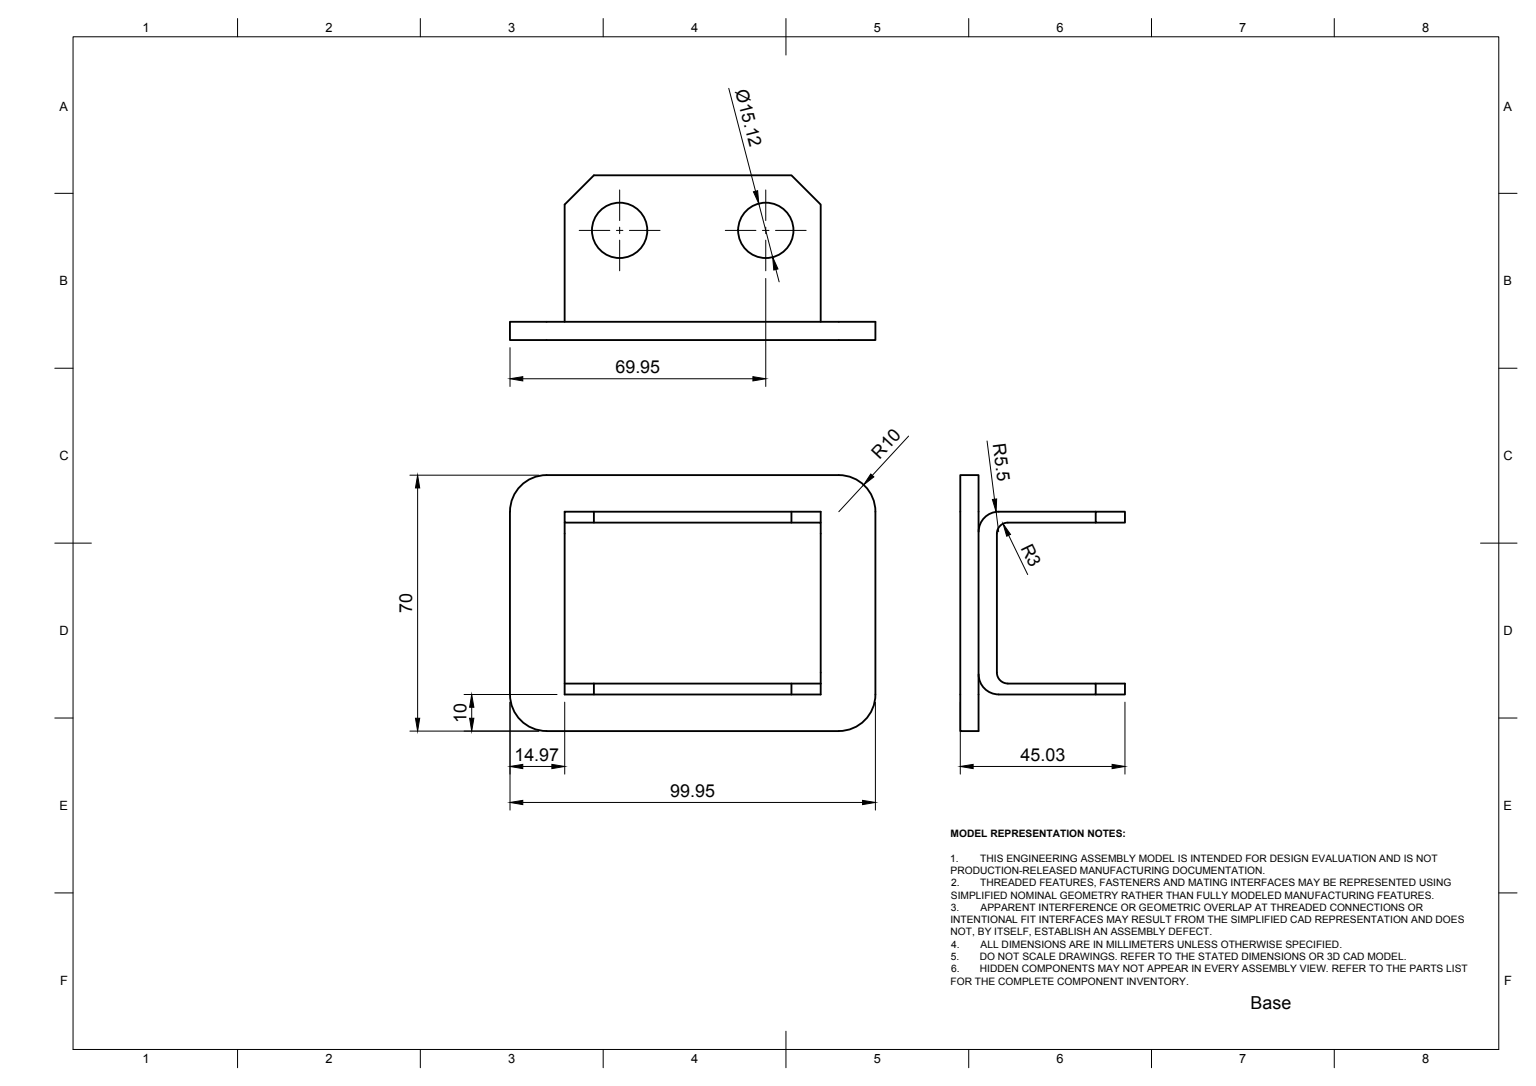
ISO-10303-21;
HEADER;
/* Generated by software containing ST-Developer
 * from STEP Tools, Inc. (www.steptools.com) 
 */

FILE_DESCRIPTION(
/* description */ (''),
/* implementation_level */ '2;1');

FILE_NAME(
/* name */ 'Base.step',
/* time_stamp */ '2026-10-06T13:41:14-07:00',
/* author */ (''),
/* organization */ (''),
/* preprocessor_version */ 'ST-DEVELOPER v20.2',
/* originating_system */ 'Autodesk Translation Framework v15.15.0.0',
/* authorisation */ '');

FILE_SCHEMA (('AUTOMOTIVE_DESIGN { 1 0 10303 214 3 1 1 }'));
ENDSEC;

DATA;
#10=MECHANICAL_DESIGN_GEOMETRIC_PRESENTATION_REPRESENTATION('',(#1960),#279266);
#1942=SHAPE_REPRESENTATION_RELATIONSHIP('SRR','None',#279301,#1951);
#1951=ADVANCED_BREP_SHAPE_REPRESENTATION('',(#1969),#279257);
#1960=STYLED_ITEM('',(#279355),#1969);
#1969=MANIFOLD_SOLID_BREP('Body1',#14938);
#1978=FACE_BOUND('',#2587,.T.);
#1979=FACE_BOUND('',#2588,.T.);
#1980=FACE_BOUND('',#2591,.T.);
#1981=FACE_BOUND('',#2592,.T.);
#1982=FACE_BOUND('',#2604,.T.);
#1983=FACE_BOUND('',#2609,.T.);
#1984=FACE_BOUND('',#2610,.T.);
#1985=FACE_BOUND('',#2613,.T.);
#1986=FACE_BOUND('',#2614,.T.);
#2024=PLANE('',#15055);
#2025=PLANE('',#15059);
#2026=PLANE('',#15063);
#2027=PLANE('',#15068);
#2028=PLANE('',#15071);
#2029=PLANE('',#15072);
#2030=PLANE('',#15076);
#2031=PLANE('',#15077);
#2032=PLANE('',#15083);
#2033=PLANE('',#15087);
#2034=PLANE('',#15088);
#2035=PLANE('',#15089);
#2036=PLANE('',#15090);
#2037=PLANE('',#15093);
#2038=PLANE('',#15097);
#2039=PLANE('',#15099);
#2040=PLANE('',#15101);
#2041=PLANE('',#15102);
#2042=PLANE('',#15103);
#2110=FACE_OUTER_BOUND('',#2580,.T.);
#2111=FACE_OUTER_BOUND('',#2581,.T.);
#2112=FACE_OUTER_BOUND('',#2582,.T.);
#2113=FACE_OUTER_BOUND('',#2583,.T.);
#2114=FACE_OUTER_BOUND('',#2584,.T.);
#2115=FACE_OUTER_BOUND('',#2585,.T.);
#2116=FACE_OUTER_BOUND('',#2586,.T.);
#2117=FACE_OUTER_BOUND('',#2589,.T.);
#2118=FACE_OUTER_BOUND('',#2590,.T.);
#2119=FACE_OUTER_BOUND('',#2593,.T.);
#2120=FACE_OUTER_BOUND('',#2594,.T.);
#2121=FACE_OUTER_BOUND('',#2595,.T.);
#2122=FACE_OUTER_BOUND('',#2596,.T.);
#2123=FACE_OUTER_BOUND('',#2597,.T.);
#2124=FACE_OUTER_BOUND('',#2598,.T.);
#2125=FACE_OUTER_BOUND('',#2599,.T.);
#2126=FACE_OUTER_BOUND('',#2600,.T.);
#2127=FACE_OUTER_BOUND('',#2601,.T.);
#2128=FACE_OUTER_BOUND('',#2602,.T.);
#2129=FACE_OUTER_BOUND('',#2603,.T.);
#2130=FACE_OUTER_BOUND('',#2605,.T.);
#2131=FACE_OUTER_BOUND('',#2606,.T.);
#2132=FACE_OUTER_BOUND('',#2607,.T.);
#2133=FACE_OUTER_BOUND('',#2608,.T.);
#2134=FACE_OUTER_BOUND('',#2611,.T.);
#2135=FACE_OUTER_BOUND('',#2612,.T.);
#2136=FACE_OUTER_BOUND('',#2615,.T.);
#2137=FACE_OUTER_BOUND('',#2616,.T.);
#2138=FACE_OUTER_BOUND('',#2617,.T.);
#2139=FACE_OUTER_BOUND('',#2618,.T.);
#2140=FACE_OUTER_BOUND('',#2619,.T.);
#2580=EDGE_LOOP('',(#8972,#8973,#8974,#8975));
#2581=EDGE_LOOP('',(#8976,#8977,#8978,#8979));
#2582=EDGE_LOOP('',(#8980,#8981,#8982,#8983));
#2583=EDGE_LOOP('',(#8984,#8985,#8986,#8987));
#2584=EDGE_LOOP('',(#8988,#8989,#8990,#8991));
#2585=EDGE_LOOP('',(#8992,#8993,#8994,#8995));
#2586=EDGE_LOOP('',(#8996,#8997,#8998,#8999,#9000,#9001));
#2587=EDGE_LOOP('',(#9002));
#2588=EDGE_LOOP('',(#9003));
#2589=EDGE_LOOP('',(#9004,#9005,#9006,#9007));
#2590=EDGE_LOOP('',(#9008,#9009,#9010,#9011,#9012,#9013));
#2591=EDGE_LOOP('',(#9014));
#2592=EDGE_LOOP('',(#9015));
#2593=EDGE_LOOP('',(#9016,#9017,#9018,#9019));
#2594=EDGE_LOOP('',(#9020,#9021,#9022,#9023));
#2595=EDGE_LOOP('',(#9024,#9025,#9026,#9027));
#2596=EDGE_LOOP('',(#9028,#9029,#9030,#9031));
#2597=EDGE_LOOP('',(#9032,#9033,#9034,#9035));
#2598=EDGE_LOOP('',(#9036,#9037,#9038,#9039,#9040,#9041,#9042,#9043,#9044,
#9045,#9046,#9047));
#2599=EDGE_LOOP('',(#9048,#9049,#9050,#9051));
#2600=EDGE_LOOP('',(#9052,#9053,#9054,#9055));
#2601=EDGE_LOOP('',(#9056,#9057,#9058,#9059));
#2602=EDGE_LOOP('',(#9060,#9061,#9062,#9063));
#2603=EDGE_LOOP('',(#9064,#9065,#9066,#9067,#9068,#9069,#9070,#9071));
#2604=EDGE_LOOP('',(#9072,#9073,#9074,#9075));
#2605=EDGE_LOOP('',(#9076,#9077,#9078,#9079));
#2606=EDGE_LOOP('',(#9080,#9081,#9082,#9083,#9084,#9085,#9086,#9087));
#2607=EDGE_LOOP('',(#9088,#9089,#9090,#9091));
#2608=EDGE_LOOP('',(#9092,#9093,#9094,#9095,#9096,#9097));
#2609=EDGE_LOOP('',(#9098));
#2610=EDGE_LOOP('',(#9099));
#2611=EDGE_LOOP('',(#9100,#9101,#9102,#9103));
#2612=EDGE_LOOP('',(#9104,#9105,#9106,#9107,#9108,#9109));
#2613=EDGE_LOOP('',(#9110));
#2614=EDGE_LOOP('',(#9111));
#2615=EDGE_LOOP('',(#9112,#9113,#9114,#9115,#9116,#9117,#9118,#9119,#9120,
#9121,#9122,#9123));
#2616=EDGE_LOOP('',(#9124,#9125,#9126,#9127));
#2617=EDGE_LOOP('',(#9128,#9129,#9130,#9131));
#2618=EDGE_LOOP('',(#9132,#9133,#9134,#9135));
#2619=EDGE_LOOP('',(#9136,#9137,#9138,#9139));
#3096=LINE('',#17463,#3624);
#3097=LINE('',#17466,#3625);
#3098=LINE('',#17471,#3626);
#3099=LINE('',#17476,#3627);
#3100=LINE('',#17478,#3628);
#3101=LINE('',#17480,#3629);
#3102=LINE('',#17481,#3630);
#3103=LINE('',#17487,#3631);
#3104=LINE('',#17490,#3632);
#3105=LINE('',#17492,#3633);
#3106=LINE('',#17493,#3634);
#3107=LINE('',#17497,#3635);
#3108=LINE('',#17501,#3636);
#3109=LINE('',#17505,#3637);
#3110=LINE('',#17507,#3638);
#3111=LINE('',#17508,#3639);
#3112=LINE('',#17509,#3640);
#3113=LINE('',#17517,#3641);
#3114=LINE('',#17520,#3642);
#3115=LINE('',#17522,#3643);
#3116=LINE('',#17524,#3644);
#3117=LINE('',#17526,#3645);
#3118=LINE('',#17527,#3646);
#3119=LINE('',#17531,#3647);
#3120=LINE('',#17533,#3648);
#3121=LINE('',#17535,#3649);
#3122=LINE('',#17541,#3650);
#3123=LINE('',#17544,#3651);
#3124=LINE('',#17546,#3652);
#3125=LINE('',#17547,#3653);
#3126=LINE('',#17553,#3654);
#3127=LINE('',#17555,#3655);
#3128=LINE('',#17557,#3656);
#3129=LINE('',#17560,#3657);
#3130=LINE('',#17561,#3658);
#3131=LINE('',#17566,#3659);
#3132=LINE('',#17570,#3660);
#3133=LINE('',#17572,#3661);
#3134=LINE('',#17573,#3662);
#3135=LINE('',#17579,#3663);
#3136=LINE('',#17582,#3664);
#3137=LINE('',#17584,#3665);
#3138=LINE('',#17585,#3666);
#3139=LINE('',#17587,#3667);
#3140=LINE('',#17589,#3668);
#3141=LINE('',#17590,#3669);
#3142=LINE('',#17592,#3670);
#3143=LINE('',#17596,#3671);
#3144=LINE('',#17599,#3672);
#3145=LINE('',#17602,#3673);
#3146=LINE('',#17604,#3674);
#3147=LINE('',#17605,#3675);
#3148=LINE('',#17611,#3676);
#3149=LINE('',#17614,#3677);
#3150=LINE('',#17616,#3678);
#3151=LINE('',#17617,#3679);
#3152=LINE('',#17621,#3680);
#3153=LINE('',#17622,#3681);
#3154=LINE('',#17624,#3682);
#3155=LINE('',#17626,#3683);
#3624=VECTOR('',#15682,10.);
#3625=VECTOR('',#15685,10.);
#3626=VECTOR('',#15690,7.55784864301595);
#3627=VECTOR('',#15695,10.);
#3628=VECTOR('',#15696,10.);
#3629=VECTOR('',#15697,9.99999999999999);
#3630=VECTOR('',#15698,10.);
#3631=VECTOR('',#15703,10.);
#3632=VECTOR('',#15706,10.);
#3633=VECTOR('',#15709,10.);
#3634=VECTOR('',#15710,10.);
#3635=VECTOR('',#15713,10.);
#3636=VECTOR('',#15716,10.);
#3637=VECTOR('',#15721,10.);
#3638=VECTOR('',#15722,10.);
#3639=VECTOR('',#15723,10.);
#3640=VECTOR('',#15724,10.);
#3641=VECTOR('',#15731,10.);
#3642=VECTOR('',#15734,10.);
#3643=VECTOR('',#15737,10.);
#3644=VECTOR('',#15738,10.);
#3645=VECTOR('',#15739,9.99999999999999);
#3646=VECTOR('',#15740,10.);
#3647=VECTOR('',#15745,7.55784864301595);
#3648=VECTOR('',#15748,10.);
#3649=VECTOR('',#15751,10.);
#3650=VECTOR('',#15756,10.);
#3651=VECTOR('',#15759,10.);
#3652=VECTOR('',#15762,10.);
#3653=VECTOR('',#15763,10.);
#3654=VECTOR('',#15768,10.);
#3655=VECTOR('',#15769,10.);
#3656=VECTOR('',#15770,10.);
#3657=VECTOR('',#15773,10.);
#3658=VECTOR('',#15774,10.);
#3659=VECTOR('',#15779,7.55784864301595);
#3660=VECTOR('',#15784,10.);
#3661=VECTOR('',#15785,9.99999999999999);
#3662=VECTOR('',#15786,10.);
#3663=VECTOR('',#15791,10.);
#3664=VECTOR('',#15794,10.);
#3665=VECTOR('',#15797,10.);
#3666=VECTOR('',#15798,10.);
#3667=VECTOR('',#15801,10.);
#3668=VECTOR('',#15802,10.);
#3669=VECTOR('',#15803,10.);
#3670=VECTOR('',#15806,10.);
#3671=VECTOR('',#15811,10.);
#3672=VECTOR('',#15814,10.);
#3673=VECTOR('',#15817,10.);
#3674=VECTOR('',#15818,10.);
#3675=VECTOR('',#15819,10.);
#3676=VECTOR('',#15826,10.);
#3677=VECTOR('',#15829,10.);
#3678=VECTOR('',#15830,9.99999999999999);
#3679=VECTOR('',#15831,10.);
#3680=VECTOR('',#15836,10.);
#3681=VECTOR('',#15837,10.);
#3682=VECTOR('',#15840,7.55784864301595);
#3683=VECTOR('',#15843,10.);
#4152=CIRCLE('',#15050,10.);
#4153=CIRCLE('',#15051,10.);
#4154=CIRCLE('',#15053,7.55784864301595);
#4155=CIRCLE('',#15054,7.55784864301595);
#4156=CIRCLE('',#15057,10.);
#4157=CIRCLE('',#15058,10.);
#4158=CIRCLE('',#15061,3.);
#4159=CIRCLE('',#15062,3.);
#4160=CIRCLE('',#15064,7.55784864301595);
#4161=CIRCLE('',#15066,5.5);
#4162=CIRCLE('',#15067,5.5);
#4163=CIRCLE('',#15069,7.55784864301595);
#4164=CIRCLE('',#15074,10.);
#4165=CIRCLE('',#15075,10.);
#4166=CIRCLE('',#15078,5.5);
#4167=CIRCLE('',#15079,3.);
#4168=CIRCLE('',#15081,7.55784864301595);
#4169=CIRCLE('',#15082,7.55784864301595);
#4170=CIRCLE('',#15085,10.);
#4171=CIRCLE('',#15086,10.);
#4172=CIRCLE('',#15092,3.);
#4173=CIRCLE('',#15094,7.55784864301595);
#4174=CIRCLE('',#15096,5.5);
#4175=CIRCLE('',#15098,7.55784864301595);
#4300=VERTEX_POINT('',#17459);
#4301=VERTEX_POINT('',#17460);
#4302=VERTEX_POINT('',#17462);
#4303=VERTEX_POINT('',#17464);
#4304=VERTEX_POINT('',#17468);
#4305=VERTEX_POINT('',#17470);
#4306=VERTEX_POINT('',#17474);
#4307=VERTEX_POINT('',#17475);
#4308=VERTEX_POINT('',#17477);
#4309=VERTEX_POINT('',#17479);
#4310=VERTEX_POINT('',#17483);
#4311=VERTEX_POINT('',#17484);
#4312=VERTEX_POINT('',#17486);
#4313=VERTEX_POINT('',#17488);
#4314=VERTEX_POINT('',#17495);
#4315=VERTEX_POINT('',#17496);
#4316=VERTEX_POINT('',#17498);
#4317=VERTEX_POINT('',#17500);
#4318=VERTEX_POINT('',#17504);
#4319=VERTEX_POINT('',#17506);
#4320=VERTEX_POINT('',#17510);
#4321=VERTEX_POINT('',#17513);
#4322=VERTEX_POINT('',#17514);
#4323=VERTEX_POINT('',#17516);
#4324=VERTEX_POINT('',#17518);
#4325=VERTEX_POINT('',#17523);
#4326=VERTEX_POINT('',#17525);
#4327=VERTEX_POINT('',#17528);
#4328=VERTEX_POINT('',#17537);
#4329=VERTEX_POINT('',#17538);
#4330=VERTEX_POINT('',#17540);
#4331=VERTEX_POINT('',#17542);
#4332=VERTEX_POINT('',#17549);
#4333=VERTEX_POINT('',#17550);
#4334=VERTEX_POINT('',#17552);
#4335=VERTEX_POINT('',#17554);
#4336=VERTEX_POINT('',#17556);
#4337=VERTEX_POINT('',#17558);
#4338=VERTEX_POINT('',#17563);
#4339=VERTEX_POINT('',#17565);
#4340=VERTEX_POINT('',#17569);
#4341=VERTEX_POINT('',#17571);
#4342=VERTEX_POINT('',#17575);
#4343=VERTEX_POINT('',#17576);
#4344=VERTEX_POINT('',#17578);
#4345=VERTEX_POINT('',#17580);
#4346=VERTEX_POINT('',#17588);
#4347=VERTEX_POINT('',#17595);
#4348=VERTEX_POINT('',#17597);
#4349=VERTEX_POINT('',#17601);
#4350=VERTEX_POINT('',#17603);
#4351=VERTEX_POINT('',#17606);
#4352=VERTEX_POINT('',#17609);
#4353=VERTEX_POINT('',#17613);
#4354=VERTEX_POINT('',#17615);
#4355=VERTEX_POINT('',#17618);
#6411=EDGE_CURVE('',#4300,#4301,#4152,.T.);
#6412=EDGE_CURVE('',#4301,#4302,#3096,.T.);
#6413=EDGE_CURVE('',#4302,#4303,#4153,.T.);
#6414=EDGE_CURVE('',#4303,#4300,#3097,.T.);
#6415=EDGE_CURVE('',#4304,#4304,#4154,.T.);
#6416=EDGE_CURVE('',#4304,#4305,#3098,.T.);
#6417=EDGE_CURVE('',#4305,#4305,#4155,.T.);
#6418=EDGE_CURVE('',#4306,#4307,#3099,.T.);
#6419=EDGE_CURVE('',#4307,#4308,#3100,.T.);
#6420=EDGE_CURVE('',#4309,#4308,#3101,.T.);
#6421=EDGE_CURVE('',#4306,#4309,#3102,.T.);
#6422=EDGE_CURVE('',#4310,#4311,#4156,.T.);
#6423=EDGE_CURVE('',#4312,#4310,#3103,.T.);
#6424=EDGE_CURVE('',#4313,#4312,#4157,.T.);
#6425=EDGE_CURVE('',#4311,#4313,#3104,.T.);
#6426=EDGE_CURVE('',#4313,#4302,#3105,.T.);
#6427=EDGE_CURVE('',#4311,#4301,#3106,.T.);
#6428=EDGE_CURVE('',#4314,#4315,#3107,.T.);
#6429=EDGE_CURVE('',#4314,#4316,#4158,.T.);
#6430=EDGE_CURVE('',#4317,#4316,#3108,.T.);
#6431=EDGE_CURVE('',#4315,#4317,#4159,.T.);
#6432=EDGE_CURVE('',#4315,#4318,#3109,.T.);
#6433=EDGE_CURVE('',#4318,#4319,#3110,.T.);
#6434=EDGE_CURVE('',#4307,#4319,#3111,.T.);
#6435=EDGE_CURVE('',#4314,#4306,#3112,.T.);
#6436=EDGE_CURVE('',#4320,#4320,#4160,.T.);
#6437=EDGE_CURVE('',#4321,#4322,#4161,.T.);
#6438=EDGE_CURVE('',#4323,#4321,#3113,.T.);
#6439=EDGE_CURVE('',#4323,#4324,#4162,.T.);
#6440=EDGE_CURVE('',#4322,#4324,#3114,.T.);
#6441=EDGE_CURVE('',#4324,#4309,#3115,.T.);
#6442=EDGE_CURVE('',#4325,#4308,#3116,.T.);
#6443=EDGE_CURVE('',#4326,#4325,#3117,.T.);
#6444=EDGE_CURVE('',#4322,#4326,#3118,.T.);
#6445=EDGE_CURVE('',#4327,#4327,#4163,.T.);
#6446=EDGE_CURVE('',#4327,#4320,#3119,.T.);
#6447=EDGE_CURVE('',#4319,#4325,#3120,.T.);
#6448=EDGE_CURVE('',#4318,#4326,#3121,.T.);
#6449=EDGE_CURVE('',#4328,#4329,#4164,.T.);
#6450=EDGE_CURVE('',#4330,#4328,#3122,.T.);
#6451=EDGE_CURVE('',#4331,#4330,#4165,.T.);
#6452=EDGE_CURVE('',#4329,#4331,#3123,.T.);
#6453=EDGE_CURVE('',#4300,#4328,#3124,.T.);
#6454=EDGE_CURVE('',#4303,#4330,#3125,.T.);
#6455=EDGE_CURVE('',#4332,#4333,#4166,.T.);
#6456=EDGE_CURVE('',#4333,#4334,#3126,.T.);
#6457=EDGE_CURVE('',#4335,#4334,#3127,.T.);
#6458=EDGE_CURVE('',#4336,#4335,#3128,.T.);
#6459=EDGE_CURVE('',#4336,#4337,#4167,.T.);
#6460=EDGE_CURVE('',#4337,#4316,#3129,.T.);
#6461=EDGE_CURVE('',#4323,#4332,#3130,.T.);
#6462=EDGE_CURVE('',#4338,#4338,#4168,.T.);
#6463=EDGE_CURVE('',#4338,#4339,#3131,.T.);
#6464=EDGE_CURVE('',#4339,#4339,#4169,.T.);
#6465=EDGE_CURVE('',#4335,#4340,#3132,.T.);
#6466=EDGE_CURVE('',#4334,#4341,#3133,.T.);
#6467=EDGE_CURVE('',#4340,#4341,#3134,.T.);
#6468=EDGE_CURVE('',#4342,#4343,#4170,.T.);
#6469=EDGE_CURVE('',#4343,#4344,#3135,.T.);
#6470=EDGE_CURVE('',#4344,#4345,#4171,.T.);
#6471=EDGE_CURVE('',#4345,#4342,#3136,.T.);
#6472=EDGE_CURVE('',#4343,#4329,#3137,.T.);
#6473=EDGE_CURVE('',#4344,#4331,#3138,.T.);
#6474=EDGE_CURVE('',#4342,#4310,#3139,.T.);
#6475=EDGE_CURVE('',#4346,#4321,#3140,.T.);
#6476=EDGE_CURVE('',#4332,#4346,#3141,.T.);
#6477=EDGE_CURVE('',#4345,#4312,#3142,.T.);
#6478=EDGE_CURVE('',#4336,#4347,#3143,.T.);
#6479=EDGE_CURVE('',#4347,#4348,#4172,.T.);
#6480=EDGE_CURVE('',#4348,#4337,#3144,.T.);
#6481=EDGE_CURVE('',#4340,#4349,#3145,.T.);
#6482=EDGE_CURVE('',#4350,#4349,#3146,.T.);
#6483=EDGE_CURVE('',#4347,#4350,#3147,.T.);
#6484=EDGE_CURVE('',#4351,#4351,#4173,.T.);
#6485=EDGE_CURVE('',#4346,#4352,#4174,.T.);
#6486=EDGE_CURVE('',#4352,#4333,#3148,.T.);
#6487=EDGE_CURVE('',#4352,#4353,#3149,.T.);
#6488=EDGE_CURVE('',#4353,#4354,#3150,.T.);
#6489=EDGE_CURVE('',#4354,#4341,#3151,.T.);
#6490=EDGE_CURVE('',#4355,#4355,#4175,.T.);
#6491=EDGE_CURVE('',#4348,#4317,#3152,.T.);
#6492=EDGE_CURVE('',#4350,#4353,#3153,.T.);
#6493=EDGE_CURVE('',#4351,#4355,#3154,.T.);
#6494=EDGE_CURVE('',#4349,#4354,#3155,.T.);
#8972=ORIENTED_EDGE('',*,*,#6411,.T.);
#8973=ORIENTED_EDGE('',*,*,#6412,.T.);
#8974=ORIENTED_EDGE('',*,*,#6413,.T.);
#8975=ORIENTED_EDGE('',*,*,#6414,.T.);
#8976=ORIENTED_EDGE('',*,*,#6415,.T.);
#8977=ORIENTED_EDGE('',*,*,#6416,.T.);
#8978=ORIENTED_EDGE('',*,*,#6417,.F.);
#8979=ORIENTED_EDGE('',*,*,#6416,.F.);
#8980=ORIENTED_EDGE('',*,*,#6418,.T.);
#8981=ORIENTED_EDGE('',*,*,#6419,.T.);
#8982=ORIENTED_EDGE('',*,*,#6420,.F.);
#8983=ORIENTED_EDGE('',*,*,#6421,.F.);
#8984=ORIENTED_EDGE('',*,*,#6422,.F.);
#8985=ORIENTED_EDGE('',*,*,#6423,.F.);
#8986=ORIENTED_EDGE('',*,*,#6424,.F.);
#8987=ORIENTED_EDGE('',*,*,#6425,.F.);
#8988=ORIENTED_EDGE('',*,*,#6425,.T.);
#8989=ORIENTED_EDGE('',*,*,#6426,.T.);
#8990=ORIENTED_EDGE('',*,*,#6412,.F.);
#8991=ORIENTED_EDGE('',*,*,#6427,.F.);
#8992=ORIENTED_EDGE('',*,*,#6428,.F.);
#8993=ORIENTED_EDGE('',*,*,#6429,.T.);
#8994=ORIENTED_EDGE('',*,*,#6430,.F.);
#8995=ORIENTED_EDGE('',*,*,#6431,.F.);
#8996=ORIENTED_EDGE('',*,*,#6428,.T.);
#8997=ORIENTED_EDGE('',*,*,#6432,.T.);
#8998=ORIENTED_EDGE('',*,*,#6433,.T.);
#8999=ORIENTED_EDGE('',*,*,#6434,.F.);
#9000=ORIENTED_EDGE('',*,*,#6418,.F.);
#9001=ORIENTED_EDGE('',*,*,#6435,.F.);
#9002=ORIENTED_EDGE('',*,*,#6415,.F.);
#9003=ORIENTED_EDGE('',*,*,#6436,.T.);
#9004=ORIENTED_EDGE('',*,*,#6437,.F.);
#9005=ORIENTED_EDGE('',*,*,#6438,.F.);
#9006=ORIENTED_EDGE('',*,*,#6439,.T.);
#9007=ORIENTED_EDGE('',*,*,#6440,.F.);
#9008=ORIENTED_EDGE('',*,*,#6440,.T.);
#9009=ORIENTED_EDGE('',*,*,#6441,.T.);
#9010=ORIENTED_EDGE('',*,*,#6420,.T.);
#9011=ORIENTED_EDGE('',*,*,#6442,.F.);
#9012=ORIENTED_EDGE('',*,*,#6443,.F.);
#9013=ORIENTED_EDGE('',*,*,#6444,.F.);
#9014=ORIENTED_EDGE('',*,*,#6417,.T.);
#9015=ORIENTED_EDGE('',*,*,#6445,.F.);
#9016=ORIENTED_EDGE('',*,*,#6445,.T.);
#9017=ORIENTED_EDGE('',*,*,#6446,.T.);
#9018=ORIENTED_EDGE('',*,*,#6436,.F.);
#9019=ORIENTED_EDGE('',*,*,#6446,.F.);
#9020=ORIENTED_EDGE('',*,*,#6434,.T.);
#9021=ORIENTED_EDGE('',*,*,#6447,.T.);
#9022=ORIENTED_EDGE('',*,*,#6442,.T.);
#9023=ORIENTED_EDGE('',*,*,#6419,.F.);
#9024=ORIENTED_EDGE('',*,*,#6433,.F.);
#9025=ORIENTED_EDGE('',*,*,#6448,.T.);
#9026=ORIENTED_EDGE('',*,*,#6443,.T.);
#9027=ORIENTED_EDGE('',*,*,#6447,.F.);
#9028=ORIENTED_EDGE('',*,*,#6449,.F.);
#9029=ORIENTED_EDGE('',*,*,#6450,.F.);
#9030=ORIENTED_EDGE('',*,*,#6451,.F.);
#9031=ORIENTED_EDGE('',*,*,#6452,.F.);
#9032=ORIENTED_EDGE('',*,*,#6450,.T.);
#9033=ORIENTED_EDGE('',*,*,#6453,.F.);
#9034=ORIENTED_EDGE('',*,*,#6414,.F.);
#9035=ORIENTED_EDGE('',*,*,#6454,.T.);
#9036=ORIENTED_EDGE('',*,*,#6455,.T.);
#9037=ORIENTED_EDGE('',*,*,#6456,.T.);
#9038=ORIENTED_EDGE('',*,*,#6457,.F.);
#9039=ORIENTED_EDGE('',*,*,#6458,.F.);
#9040=ORIENTED_EDGE('',*,*,#6459,.T.);
#9041=ORIENTED_EDGE('',*,*,#6460,.T.);
#9042=ORIENTED_EDGE('',*,*,#6429,.F.);
#9043=ORIENTED_EDGE('',*,*,#6435,.T.);
#9044=ORIENTED_EDGE('',*,*,#6421,.T.);
#9045=ORIENTED_EDGE('',*,*,#6441,.F.);
#9046=ORIENTED_EDGE('',*,*,#6439,.F.);
#9047=ORIENTED_EDGE('',*,*,#6461,.T.);
#9048=ORIENTED_EDGE('',*,*,#6462,.T.);
#9049=ORIENTED_EDGE('',*,*,#6463,.T.);
#9050=ORIENTED_EDGE('',*,*,#6464,.F.);
#9051=ORIENTED_EDGE('',*,*,#6463,.F.);
#9052=ORIENTED_EDGE('',*,*,#6465,.F.);
#9053=ORIENTED_EDGE('',*,*,#6457,.T.);
#9054=ORIENTED_EDGE('',*,*,#6466,.T.);
#9055=ORIENTED_EDGE('',*,*,#6467,.F.);
#9056=ORIENTED_EDGE('',*,*,#6468,.T.);
#9057=ORIENTED_EDGE('',*,*,#6469,.T.);
#9058=ORIENTED_EDGE('',*,*,#6470,.T.);
#9059=ORIENTED_EDGE('',*,*,#6471,.T.);
#9060=ORIENTED_EDGE('',*,*,#6469,.F.);
#9061=ORIENTED_EDGE('',*,*,#6472,.T.);
#9062=ORIENTED_EDGE('',*,*,#6452,.T.);
#9063=ORIENTED_EDGE('',*,*,#6473,.F.);
#9064=ORIENTED_EDGE('',*,*,#6453,.T.);
#9065=ORIENTED_EDGE('',*,*,#6449,.T.);
#9066=ORIENTED_EDGE('',*,*,#6472,.F.);
#9067=ORIENTED_EDGE('',*,*,#6468,.F.);
#9068=ORIENTED_EDGE('',*,*,#6474,.T.);
#9069=ORIENTED_EDGE('',*,*,#6422,.T.);
#9070=ORIENTED_EDGE('',*,*,#6427,.T.);
#9071=ORIENTED_EDGE('',*,*,#6411,.F.);
#9072=ORIENTED_EDGE('',*,*,#6461,.F.);
#9073=ORIENTED_EDGE('',*,*,#6438,.T.);
#9074=ORIENTED_EDGE('',*,*,#6475,.F.);
#9075=ORIENTED_EDGE('',*,*,#6476,.F.);
#9076=ORIENTED_EDGE('',*,*,#6471,.F.);
#9077=ORIENTED_EDGE('',*,*,#6477,.T.);
#9078=ORIENTED_EDGE('',*,*,#6423,.T.);
#9079=ORIENTED_EDGE('',*,*,#6474,.F.);
#9080=ORIENTED_EDGE('',*,*,#6470,.F.);
#9081=ORIENTED_EDGE('',*,*,#6473,.T.);
#9082=ORIENTED_EDGE('',*,*,#6451,.T.);
#9083=ORIENTED_EDGE('',*,*,#6454,.F.);
#9084=ORIENTED_EDGE('',*,*,#6413,.F.);
#9085=ORIENTED_EDGE('',*,*,#6426,.F.);
#9086=ORIENTED_EDGE('',*,*,#6424,.T.);
#9087=ORIENTED_EDGE('',*,*,#6477,.F.);
#9088=ORIENTED_EDGE('',*,*,#6478,.T.);
#9089=ORIENTED_EDGE('',*,*,#6479,.T.);
#9090=ORIENTED_EDGE('',*,*,#6480,.T.);
#9091=ORIENTED_EDGE('',*,*,#6459,.F.);
#9092=ORIENTED_EDGE('',*,*,#6478,.F.);
#9093=ORIENTED_EDGE('',*,*,#6458,.T.);
#9094=ORIENTED_EDGE('',*,*,#6465,.T.);
#9095=ORIENTED_EDGE('',*,*,#6481,.T.);
#9096=ORIENTED_EDGE('',*,*,#6482,.F.);
#9097=ORIENTED_EDGE('',*,*,#6483,.F.);
#9098=ORIENTED_EDGE('',*,*,#6464,.T.);
#9099=ORIENTED_EDGE('',*,*,#6484,.F.);
#9100=ORIENTED_EDGE('',*,*,#6485,.T.);
#9101=ORIENTED_EDGE('',*,*,#6486,.T.);
#9102=ORIENTED_EDGE('',*,*,#6455,.F.);
#9103=ORIENTED_EDGE('',*,*,#6476,.T.);
#9104=ORIENTED_EDGE('',*,*,#6486,.F.);
#9105=ORIENTED_EDGE('',*,*,#6487,.T.);
#9106=ORIENTED_EDGE('',*,*,#6488,.T.);
#9107=ORIENTED_EDGE('',*,*,#6489,.T.);
#9108=ORIENTED_EDGE('',*,*,#6466,.F.);
#9109=ORIENTED_EDGE('',*,*,#6456,.F.);
#9110=ORIENTED_EDGE('',*,*,#6462,.F.);
#9111=ORIENTED_EDGE('',*,*,#6490,.T.);
#9112=ORIENTED_EDGE('',*,*,#6485,.F.);
#9113=ORIENTED_EDGE('',*,*,#6475,.T.);
#9114=ORIENTED_EDGE('',*,*,#6437,.T.);
#9115=ORIENTED_EDGE('',*,*,#6444,.T.);
#9116=ORIENTED_EDGE('',*,*,#6448,.F.);
#9117=ORIENTED_EDGE('',*,*,#6432,.F.);
#9118=ORIENTED_EDGE('',*,*,#6431,.T.);
#9119=ORIENTED_EDGE('',*,*,#6491,.F.);
#9120=ORIENTED_EDGE('',*,*,#6479,.F.);
#9121=ORIENTED_EDGE('',*,*,#6483,.T.);
#9122=ORIENTED_EDGE('',*,*,#6492,.T.);
#9123=ORIENTED_EDGE('',*,*,#6487,.F.);
#9124=ORIENTED_EDGE('',*,*,#6484,.T.);
#9125=ORIENTED_EDGE('',*,*,#6493,.T.);
#9126=ORIENTED_EDGE('',*,*,#6490,.F.);
#9127=ORIENTED_EDGE('',*,*,#6493,.F.);
#9128=ORIENTED_EDGE('',*,*,#6481,.F.);
#9129=ORIENTED_EDGE('',*,*,#6467,.T.);
#9130=ORIENTED_EDGE('',*,*,#6489,.F.);
#9131=ORIENTED_EDGE('',*,*,#6494,.F.);
#9132=ORIENTED_EDGE('',*,*,#6482,.T.);
#9133=ORIENTED_EDGE('',*,*,#6494,.T.);
#9134=ORIENTED_EDGE('',*,*,#6488,.F.);
#9135=ORIENTED_EDGE('',*,*,#6492,.F.);
#9136=ORIENTED_EDGE('',*,*,#6480,.F.);
#9137=ORIENTED_EDGE('',*,*,#6491,.T.);
#9138=ORIENTED_EDGE('',*,*,#6430,.T.);
#9139=ORIENTED_EDGE('',*,*,#6460,.F.);
#14094=CYLINDRICAL_SURFACE('',#15049,10.);
#14095=CYLINDRICAL_SURFACE('',#15052,7.55784864301595);
#14096=CYLINDRICAL_SURFACE('',#15056,10.);
#14097=CYLINDRICAL_SURFACE('',#15060,3.);
#14098=CYLINDRICAL_SURFACE('',#15065,5.5);
#14099=CYLINDRICAL_SURFACE('',#15070,7.55784864301595);
#14100=CYLINDRICAL_SURFACE('',#15073,10.);
#14101=CYLINDRICAL_SURFACE('',#15080,7.55784864301595);
#14102=CYLINDRICAL_SURFACE('',#15084,10.);
#14103=CYLINDRICAL_SURFACE('',#15091,3.);
#14104=CYLINDRICAL_SURFACE('',#15095,5.5);
#14105=CYLINDRICAL_SURFACE('',#15100,7.55784864301595);
#14468=ADVANCED_FACE('',(#2110),#14094,.T.);
#14469=ADVANCED_FACE('',(#2111),#14095,.F.);
#14470=ADVANCED_FACE('',(#2112),#2024,.T.);
#14471=ADVANCED_FACE('',(#2113),#14096,.T.);
#14472=ADVANCED_FACE('',(#2114),#2025,.F.);
#14473=ADVANCED_FACE('',(#2115),#14097,.F.);
#14474=ADVANCED_FACE('',(#2116,#1978,#1979),#2026,.F.);
#14475=ADVANCED_FACE('',(#2117),#14098,.T.);
#14476=ADVANCED_FACE('',(#2118,#1980,#1981),#2027,.F.);
#14477=ADVANCED_FACE('',(#2119),#14099,.F.);
#14478=ADVANCED_FACE('',(#2120),#2028,.F.);
#14479=ADVANCED_FACE('',(#2121),#2029,.F.);
#14480=ADVANCED_FACE('',(#2122),#14100,.T.);
#14481=ADVANCED_FACE('',(#2123),#2030,.F.);
#14482=ADVANCED_FACE('',(#2124),#2031,.F.);
#14483=ADVANCED_FACE('',(#2125),#14101,.F.);
#14484=ADVANCED_FACE('',(#2126),#2032,.F.);
#14485=ADVANCED_FACE('',(#2127),#14102,.T.);
#14486=ADVANCED_FACE('',(#2128),#2033,.T.);
#14487=ADVANCED_FACE('',(#2129,#1982),#2034,.T.);
#14488=ADVANCED_FACE('',(#2130),#2035,.T.);
#14489=ADVANCED_FACE('',(#2131),#2036,.T.);
#14490=ADVANCED_FACE('',(#2132),#14103,.F.);
#14491=ADVANCED_FACE('',(#2133,#1983,#1984),#2037,.T.);
#14492=ADVANCED_FACE('',(#2134),#14104,.T.);
#14493=ADVANCED_FACE('',(#2135,#1985,#1986),#2038,.T.);
#14494=ADVANCED_FACE('',(#2136),#2039,.T.);
#14495=ADVANCED_FACE('',(#2137),#14105,.F.);
#14496=ADVANCED_FACE('',(#2138),#2040,.T.);
#14497=ADVANCED_FACE('',(#2139),#2041,.T.);
#14498=ADVANCED_FACE('',(#2140),#2042,.T.);
#14938=CLOSED_SHELL('',(#14468,#14469,#14470,#14471,#14472,#14473,#14474,
#14475,#14476,#14477,#14478,#14479,#14480,#14481,#14482,#14483,#14484,#14485,
#14486,#14487,#14488,#14489,#14490,#14491,#14492,#14493,#14494,#14495,#14496,
#14497,#14498));
#15048=AXIS2_PLACEMENT_3D('',#17457,#15676,#15677);
#15049=AXIS2_PLACEMENT_3D('',#17458,#15678,#15679);
#15050=AXIS2_PLACEMENT_3D('',#17461,#15680,#15681);
#15051=AXIS2_PLACEMENT_3D('',#17465,#15683,#15684);
#15052=AXIS2_PLACEMENT_3D('',#17467,#15686,#15687);
#15053=AXIS2_PLACEMENT_3D('',#17469,#15688,#15689);
#15054=AXIS2_PLACEMENT_3D('',#17472,#15691,#15692);
#15055=AXIS2_PLACEMENT_3D('',#17473,#15693,#15694);
#15056=AXIS2_PLACEMENT_3D('',#17482,#15699,#15700);
#15057=AXIS2_PLACEMENT_3D('',#17485,#15701,#15702);
#15058=AXIS2_PLACEMENT_3D('',#17489,#15704,#15705);
#15059=AXIS2_PLACEMENT_3D('',#17491,#15707,#15708);
#15060=AXIS2_PLACEMENT_3D('',#17494,#15711,#15712);
#15061=AXIS2_PLACEMENT_3D('',#17499,#15714,#15715);
#15062=AXIS2_PLACEMENT_3D('',#17502,#15717,#15718);
#15063=AXIS2_PLACEMENT_3D('',#17503,#15719,#15720);
#15064=AXIS2_PLACEMENT_3D('',#17511,#15725,#15726);
#15065=AXIS2_PLACEMENT_3D('',#17512,#15727,#15728);
#15066=AXIS2_PLACEMENT_3D('',#17515,#15729,#15730);
#15067=AXIS2_PLACEMENT_3D('',#17519,#15732,#15733);
#15068=AXIS2_PLACEMENT_3D('',#17521,#15735,#15736);
#15069=AXIS2_PLACEMENT_3D('',#17529,#15741,#15742);
#15070=AXIS2_PLACEMENT_3D('',#17530,#15743,#15744);
#15071=AXIS2_PLACEMENT_3D('',#17532,#15746,#15747);
#15072=AXIS2_PLACEMENT_3D('',#17534,#15749,#15750);
#15073=AXIS2_PLACEMENT_3D('',#17536,#15752,#15753);
#15074=AXIS2_PLACEMENT_3D('',#17539,#15754,#15755);
#15075=AXIS2_PLACEMENT_3D('',#17543,#15757,#15758);
#15076=AXIS2_PLACEMENT_3D('',#17545,#15760,#15761);
#15077=AXIS2_PLACEMENT_3D('',#17548,#15764,#15765);
#15078=AXIS2_PLACEMENT_3D('',#17551,#15766,#15767);
#15079=AXIS2_PLACEMENT_3D('',#17559,#15771,#15772);
#15080=AXIS2_PLACEMENT_3D('',#17562,#15775,#15776);
#15081=AXIS2_PLACEMENT_3D('',#17564,#15777,#15778);
#15082=AXIS2_PLACEMENT_3D('',#17567,#15780,#15781);
#15083=AXIS2_PLACEMENT_3D('',#17568,#15782,#15783);
#15084=AXIS2_PLACEMENT_3D('',#17574,#15787,#15788);
#15085=AXIS2_PLACEMENT_3D('',#17577,#15789,#15790);
#15086=AXIS2_PLACEMENT_3D('',#17581,#15792,#15793);
#15087=AXIS2_PLACEMENT_3D('',#17583,#15795,#15796);
#15088=AXIS2_PLACEMENT_3D('',#17586,#15799,#15800);
#15089=AXIS2_PLACEMENT_3D('',#17591,#15804,#15805);
#15090=AXIS2_PLACEMENT_3D('',#17593,#15807,#15808);
#15091=AXIS2_PLACEMENT_3D('',#17594,#15809,#15810);
#15092=AXIS2_PLACEMENT_3D('',#17598,#15812,#15813);
#15093=AXIS2_PLACEMENT_3D('',#17600,#15815,#15816);
#15094=AXIS2_PLACEMENT_3D('',#17607,#15820,#15821);
#15095=AXIS2_PLACEMENT_3D('',#17608,#15822,#15823);
#15096=AXIS2_PLACEMENT_3D('',#17610,#15824,#15825);
#15097=AXIS2_PLACEMENT_3D('',#17612,#15827,#15828);
#15098=AXIS2_PLACEMENT_3D('',#17619,#15832,#15833);
#15099=AXIS2_PLACEMENT_3D('',#17620,#15834,#15835);
#15100=AXIS2_PLACEMENT_3D('',#17623,#15838,#15839);
#15101=AXIS2_PLACEMENT_3D('',#17625,#15841,#15842);
#15102=AXIS2_PLACEMENT_3D('',#17627,#15844,#15845);
#15103=AXIS2_PLACEMENT_3D('',#17628,#15846,#15847);
#15676=DIRECTION('axis',(0.,0.,1.));
#15677=DIRECTION('refdir',(1.,0.,0.));
#15678=DIRECTION('center_axis',(0.,0.,1.));
#15679=DIRECTION('ref_axis',(-0.707106781186548,0.707106781186548,0.));
#15680=DIRECTION('center_axis',(0.,0.,-1.));
#15681=DIRECTION('ref_axis',(-0.707106781186548,0.707106781186548,0.));
#15682=DIRECTION('',(0.,0.,-1.));
#15683=DIRECTION('center_axis',(0.,0.,1.));
#15684=DIRECTION('ref_axis',(-0.707106781186548,0.707106781186548,0.));
#15685=DIRECTION('',(0.,0.,1.));
#15686=DIRECTION('center_axis',(0.,1.,0.));
#15687=DIRECTION('ref_axis',(-1.,0.,0.));
#15688=DIRECTION('center_axis',(0.,-1.,0.));
#15689=DIRECTION('ref_axis',(-1.,0.,0.));
#15690=DIRECTION('',(0.,1.,0.));
#15691=DIRECTION('center_axis',(0.,-1.,0.));
#15692=DIRECTION('ref_axis',(-1.,0.,0.));
#15693=DIRECTION('center_axis',(-0.707106781186548,0.,0.707106781186548));
#15694=DIRECTION('ref_axis',(0.707106781186548,0.,0.707106781186548));
#15695=DIRECTION('',(0.707106781186547,0.,0.707106781186547));
#15696=DIRECTION('',(0.,1.,0.));
#15697=DIRECTION('',(0.707106781186547,0.,0.707106781186547));
#15698=DIRECTION('',(0.,1.,0.));
#15699=DIRECTION('center_axis',(0.,0.,-1.));
#15700=DIRECTION('ref_axis',(0.707106781186548,0.707106781186548,0.));
#15701=DIRECTION('center_axis',(0.,0.,1.));
#15702=DIRECTION('ref_axis',(0.707106781186548,0.707106781186548,0.));
#15703=DIRECTION('',(0.,0.,1.));
#15704=DIRECTION('center_axis',(0.,0.,-1.));
#15705=DIRECTION('ref_axis',(0.707106781186548,0.707106781186548,0.));
#15706=DIRECTION('',(0.,0.,-1.));
#15707=DIRECTION('center_axis',(0.,-1.,0.));
#15708=DIRECTION('ref_axis',(0.,0.,-1.));
#15709=DIRECTION('',(-1.,0.,0.));
#15710=DIRECTION('',(-1.,0.,0.));
#15711=DIRECTION('center_axis',(-1.,0.,0.));
#15712=DIRECTION('ref_axis',(0.,0.707106781186548,-0.707106781186547));
#15713=DIRECTION('',(1.,0.,0.));
#15714=DIRECTION('center_axis',(-1.,0.,0.));
#15715=DIRECTION('ref_axis',(0.,0.707106781186548,-0.707106781186547));
#15716=DIRECTION('',(-1.,0.,0.));
#15717=DIRECTION('center_axis',(-1.,0.,0.));
#15718=DIRECTION('ref_axis',(0.,0.707106781186548,-0.707106781186547));
#15719=DIRECTION('center_axis',(0.,1.,0.));
#15720=DIRECTION('ref_axis',(1.,0.,0.));
#15721=DIRECTION('',(0.,0.,1.));
#15722=DIRECTION('',(-0.707106781186547,0.,0.707106781186547));
#15723=DIRECTION('',(1.,0.,0.));
#15724=DIRECTION('',(0.,0.,1.));
#15725=DIRECTION('center_axis',(0.,1.,0.));
#15726=DIRECTION('ref_axis',(1.,0.,0.));
#15727=DIRECTION('center_axis',(-1.,0.,0.));
#15728=DIRECTION('ref_axis',(0.,0.707106781186548,-0.707106781186547));
#15729=DIRECTION('center_axis',(1.,0.,0.));
#15730=DIRECTION('ref_axis',(0.,0.707106781186548,-0.707106781186547));
#15731=DIRECTION('',(1.,0.,0.));
#15732=DIRECTION('center_axis',(1.,0.,0.));
#15733=DIRECTION('ref_axis',(0.,0.707106781186548,-0.707106781186547));
#15734=DIRECTION('',(-1.,0.,0.));
#15735=DIRECTION('center_axis',(0.,-1.,0.));
#15736=DIRECTION('ref_axis',(0.,0.,-1.));
#15737=DIRECTION('',(0.,0.,1.));
#15738=DIRECTION('',(-1.,0.,0.));
#15739=DIRECTION('',(-0.707106781186547,0.,0.707106781186547));
#15740=DIRECTION('',(0.,0.,1.));
#15741=DIRECTION('center_axis',(0.,1.,0.));
#15742=DIRECTION('ref_axis',(1.,0.,0.));
#15743=DIRECTION('center_axis',(0.,-1.,0.));
#15744=DIRECTION('ref_axis',(1.,0.,0.));
#15745=DIRECTION('',(0.,-1.,0.));
#15746=DIRECTION('center_axis',(0.,0.,-1.));
#15747=DIRECTION('ref_axis',(-1.,0.,0.));
#15748=DIRECTION('',(0.,1.,0.));
#15749=DIRECTION('center_axis',(-0.707106781186548,0.,-0.707106781186548));
#15750=DIRECTION('ref_axis',(-0.707106781186548,0.,0.707106781186548));
#15751=DIRECTION('',(0.,1.,0.));
#15752=DIRECTION('center_axis',(0.,0.,-1.));
#15753=DIRECTION('ref_axis',(-0.707106781186548,-0.707106781186548,0.));
#15754=DIRECTION('center_axis',(0.,0.,1.));
#15755=DIRECTION('ref_axis',(-0.707106781186548,-0.707106781186548,0.));
#15756=DIRECTION('',(0.,0.,1.));
#15757=DIRECTION('center_axis',(0.,0.,-1.));
#15758=DIRECTION('ref_axis',(-0.707106781186548,-0.707106781186548,0.));
#15759=DIRECTION('',(0.,0.,-1.));
#15760=DIRECTION('center_axis',(1.,0.,0.));
#15761=DIRECTION('ref_axis',(0.,0.,1.));
#15762=DIRECTION('',(0.,-1.,0.));
#15763=DIRECTION('',(0.,-1.,0.));
#15764=DIRECTION('center_axis',(1.,0.,0.));
#15765=DIRECTION('ref_axis',(0.,0.,1.));
#15766=DIRECTION('center_axis',(-1.,0.,0.));
#15767=DIRECTION('ref_axis',(0.,-0.707106781186548,-0.707106781186547));
#15768=DIRECTION('',(0.,0.,1.));
#15769=DIRECTION('',(0.,-1.,0.));
#15770=DIRECTION('',(0.,0.,1.));
#15771=DIRECTION('center_axis',(1.,0.,0.));
#15772=DIRECTION('ref_axis',(0.,-0.707106781186548,-0.707106781186547));
#15773=DIRECTION('',(0.,1.,0.));
#15774=DIRECTION('',(0.,-1.,0.));
#15775=DIRECTION('center_axis',(0.,1.,0.));
#15776=DIRECTION('ref_axis',(-1.,0.,0.));
#15777=DIRECTION('center_axis',(0.,-1.,0.));
#15778=DIRECTION('ref_axis',(-1.,0.,0.));
#15779=DIRECTION('',(0.,1.,0.));
#15780=DIRECTION('center_axis',(0.,-1.,0.));
#15781=DIRECTION('ref_axis',(-1.,0.,0.));
#15782=DIRECTION('center_axis',(0.707106781186548,0.,-0.707106781186548));
#15783=DIRECTION('ref_axis',(0.707106781186548,0.,0.707106781186548));
#15784=DIRECTION('',(0.707106781186547,0.,0.707106781186547));
#15785=DIRECTION('',(0.707106781186547,0.,0.707106781186547));
#15786=DIRECTION('',(0.,-1.,0.));
#15787=DIRECTION('center_axis',(0.,0.,1.));
#15788=DIRECTION('ref_axis',(0.707106781186548,-0.707106781186548,0.));
#15789=DIRECTION('center_axis',(0.,0.,-1.));
#15790=DIRECTION('ref_axis',(0.707106781186548,-0.707106781186548,0.));
#15791=DIRECTION('',(0.,0.,-1.));
#15792=DIRECTION('center_axis',(0.,0.,1.));
#15793=DIRECTION('ref_axis',(0.707106781186548,-0.707106781186548,0.));
#15794=DIRECTION('',(0.,0.,1.));
#15795=DIRECTION('center_axis',(0.,-1.,0.));
#15796=DIRECTION('ref_axis',(0.,0.,-1.));
#15797=DIRECTION('',(-1.,0.,0.));
#15798=DIRECTION('',(-1.,0.,0.));
#15799=DIRECTION('center_axis',(0.,0.,1.));
#15800=DIRECTION('ref_axis',(-1.,0.,0.));
#15801=DIRECTION('',(0.,1.,0.));
#15802=DIRECTION('',(0.,1.,0.));
#15803=DIRECTION('',(1.,0.,0.));
#15804=DIRECTION('center_axis',(1.,0.,0.));
#15805=DIRECTION('ref_axis',(0.,0.,1.));
#15806=DIRECTION('',(0.,1.,0.));
#15807=DIRECTION('center_axis',(0.,0.,-1.));
#15808=DIRECTION('ref_axis',(1.,0.,0.));
#15809=DIRECTION('center_axis',(1.,0.,0.));
#15810=DIRECTION('ref_axis',(0.,-0.707106781186548,-0.707106781186547));
#15811=DIRECTION('',(1.,0.,0.));
#15812=DIRECTION('center_axis',(1.,0.,0.));
#15813=DIRECTION('ref_axis',(0.,-0.707106781186548,-0.707106781186547));
#15814=DIRECTION('',(-1.,0.,0.));
#15815=DIRECTION('center_axis',(0.,1.,0.));
#15816=DIRECTION('ref_axis',(1.,0.,0.));
#15817=DIRECTION('',(1.,0.,0.));
#15818=DIRECTION('',(-0.707106781186547,0.,0.707106781186547));
#15819=DIRECTION('',(0.,0.,1.));
#15820=DIRECTION('center_axis',(0.,1.,0.));
#15821=DIRECTION('ref_axis',(1.,0.,0.));
#15822=DIRECTION('center_axis',(1.,0.,0.));
#15823=DIRECTION('ref_axis',(0.,-0.707106781186548,-0.707106781186547));
#15824=DIRECTION('center_axis',(-1.,0.,0.));
#15825=DIRECTION('ref_axis',(0.,-0.707106781186548,-0.707106781186547));
#15826=DIRECTION('',(-1.,0.,0.));
#15827=DIRECTION('center_axis',(0.,-1.,0.));
#15828=DIRECTION('ref_axis',(0.,0.,-1.));
#15829=DIRECTION('',(0.,0.,1.));
#15830=DIRECTION('',(-0.707106781186547,0.,0.707106781186547));
#15831=DIRECTION('',(-1.,0.,0.));
#15832=DIRECTION('center_axis',(0.,1.,0.));
#15833=DIRECTION('ref_axis',(1.,0.,0.));
#15834=DIRECTION('center_axis',(1.,0.,0.));
#15835=DIRECTION('ref_axis',(0.,0.,1.));
#15836=DIRECTION('',(0.,1.,0.));
#15837=DIRECTION('',(0.,-1.,0.));
#15838=DIRECTION('center_axis',(0.,-1.,0.));
#15839=DIRECTION('ref_axis',(1.,0.,0.));
#15840=DIRECTION('',(0.,-1.,0.));
#15841=DIRECTION('center_axis',(0.,0.,1.));
#15842=DIRECTION('ref_axis',(-1.,0.,0.));
#15843=DIRECTION('',(0.,-1.,0.));
#15844=DIRECTION('center_axis',(0.707106781186548,0.,0.707106781186548));
#15845=DIRECTION('ref_axis',(-0.707106781186548,0.,0.707106781186548));
#15846=DIRECTION('center_axis',(0.,0.,1.));
#15847=DIRECTION('ref_axis',(-1.,0.,0.));
#17457=CARTESIAN_POINT('',(0.,0.,0.));
#17458=CARTESIAN_POINT('Origin',(-39.9751670169646,25.,1.25));
#17459=CARTESIAN_POINT('',(-49.9751670169646,25.,5.));
#17460=CARTESIAN_POINT('',(-39.9751670169646,35.,5.));
#17461=CARTESIAN_POINT('Origin',(-39.9751670169646,25.,5.));
#17462=CARTESIAN_POINT('',(-39.9751670169646,35.,0.));
#17463=CARTESIAN_POINT('',(-39.9751670169646,35.,1.25));
#17464=CARTESIAN_POINT('',(-49.9751670169646,25.,0.));
#17465=CARTESIAN_POINT('Origin',(-39.9751670169646,25.,0.));
#17466=CARTESIAN_POINT('',(-49.9751670169646,25.,1.25));
#17467=CARTESIAN_POINT('Origin',(-19.9792411332937,0.,29.9773129029999));
#17468=CARTESIAN_POINT('',(-12.4213924902778,22.,29.9773129029999));
#17469=CARTESIAN_POINT('Origin',(-19.9792411332937,22.,29.9773129029999));
#17470=CARTESIAN_POINT('',(-12.4213924902778,25.,29.9773129029999));
#17471=CARTESIAN_POINT('',(-12.4213924902778,0.,29.9773129029999));
#17472=CARTESIAN_POINT('Origin',(-19.9792411332937,25.,29.9773129029999));
#17473=CARTESIAN_POINT('Origin',(-35.0075079285187,0.,37.0308437753216));
#17474=CARTESIAN_POINT('',(-35.0075079285187,22.,37.0308437753216));
#17475=CARTESIAN_POINT('',(-27.0075079285187,22.,45.0308437753216));
#17476=CARTESIAN_POINT('',(-33.010424909369,22.,39.0279267944712));
#17477=CARTESIAN_POINT('',(-27.0075079285187,25.,45.0308437753216));
#17478=CARTESIAN_POINT('',(-27.0075079285187,0.,45.0308437753216));
#17479=CARTESIAN_POINT('',(-35.0075079285187,25.,37.0308437753216));
#17480=CARTESIAN_POINT('',(-35.0075079285187,25.,37.0308437753216));
#17481=CARTESIAN_POINT('',(-35.0075079285187,0.,37.0308437753216));
#17482=CARTESIAN_POINT('Origin',(39.9751670169646,25.,1.25));
#17483=CARTESIAN_POINT('',(49.9751670169646,25.,5.));
#17484=CARTESIAN_POINT('',(39.9751670169646,35.,5.));
#17485=CARTESIAN_POINT('Origin',(39.9751670169646,25.,5.));
#17486=CARTESIAN_POINT('',(49.9751670169646,25.,0.));
#17487=CARTESIAN_POINT('',(49.9751670169646,25.,1.25));
#17488=CARTESIAN_POINT('',(39.9751670169646,35.,0.));
#17489=CARTESIAN_POINT('Origin',(39.9751670169646,25.,0.));
#17490=CARTESIAN_POINT('',(39.9751670169646,35.,1.25));
#17491=CARTESIAN_POINT('Origin',(24.9875835084823,35.,2.5));
#17492=CARTESIAN_POINT('',(0.,35.,0.));
#17493=CARTESIAN_POINT('',(0.,35.,5.));
#17494=CARTESIAN_POINT('Origin',(26.255630946389,19.,13.));
#17495=CARTESIAN_POINT('',(-35.0075079285187,22.,13.));
#17496=CARTESIAN_POINT('',(35.0075079285187,22.,13.));
#17497=CARTESIAN_POINT('',(26.255630946389,22.,13.));
#17498=CARTESIAN_POINT('',(-35.0075079285187,19.,10.));
#17499=CARTESIAN_POINT('Origin',(-35.0075079285187,19.,13.));
#17500=CARTESIAN_POINT('',(35.0075079285187,19.,10.));
#17501=CARTESIAN_POINT('',(26.255630946389,19.,10.));
#17502=CARTESIAN_POINT('Origin',(35.0075079285187,19.,13.));
#17503=CARTESIAN_POINT('Origin',(17.5037539642593,22.,27.5154218876608));
#17504=CARTESIAN_POINT('',(35.0075079285187,22.,37.0308437753216));
#17505=CARTESIAN_POINT('',(35.0075079285187,22.,18.7577109438304));
#17506=CARTESIAN_POINT('',(27.0075079285187,22.,45.0308437753216));
#17507=CARTESIAN_POINT('',(33.010424909369,22.,39.0279267944712));
#17508=CARTESIAN_POINT('',(-22.255630946389,22.,45.0308437753216));
#17509=CARTESIAN_POINT('',(-35.0075079285187,22.,18.7577109438304));
#17510=CARTESIAN_POINT('',(12.4213924902778,22.,29.9773129029999));
#17511=CARTESIAN_POINT('Origin',(19.9792411332937,22.,29.9773129029999));
#17512=CARTESIAN_POINT('Origin',(8.75187698212967,19.5,10.5));
#17513=CARTESIAN_POINT('',(35.0075079285187,19.5,5.));
#17514=CARTESIAN_POINT('',(35.0075079285187,25.,10.5));
#17515=CARTESIAN_POINT('Origin',(35.0075079285187,19.5,10.5));
#17516=CARTESIAN_POINT('',(-35.0075079285187,19.5,5.));
#17517=CARTESIAN_POINT('',(8.75187698212967,19.5,5.));
#17518=CARTESIAN_POINT('',(-35.0075079285187,25.,10.5));
#17519=CARTESIAN_POINT('Origin',(-35.0075079285187,19.5,10.5));
#17520=CARTESIAN_POINT('',(8.75187698212967,25.,10.5));
#17521=CARTESIAN_POINT('Origin',(17.5037539642593,25.,7.5));
#17522=CARTESIAN_POINT('',(-35.0075079285187,25.,5.));
#17523=CARTESIAN_POINT('',(27.0075079285187,25.,45.0308437753216));
#17524=CARTESIAN_POINT('',(27.0075079285187,25.,45.0308437753216));
#17525=CARTESIAN_POINT('',(35.0075079285187,25.,37.0308437753216));
#17526=CARTESIAN_POINT('',(35.0075079285187,25.,37.0308437753216));
#17527=CARTESIAN_POINT('',(35.0075079285187,25.,5.));
#17528=CARTESIAN_POINT('',(12.4213924902778,25.,29.9773129029999));
#17529=CARTESIAN_POINT('Origin',(19.9792411332937,25.,29.9773129029999));
#17530=CARTESIAN_POINT('Origin',(19.9792411332937,0.,29.9773129029999));
#17531=CARTESIAN_POINT('',(12.4213924902778,0.,29.9773129029999));
#17532=CARTESIAN_POINT('Origin',(27.0075079285187,0.,45.0308437753216));
#17533=CARTESIAN_POINT('',(27.0075079285187,0.,45.0308437753216));
#17534=CARTESIAN_POINT('Origin',(35.0075079285187,0.,37.0308437753216));
#17535=CARTESIAN_POINT('',(35.0075079285187,0.,37.0308437753216));
#17536=CARTESIAN_POINT('Origin',(-39.9751670169646,-25.,1.25));
#17537=CARTESIAN_POINT('',(-49.9751670169646,-25.,5.));
#17538=CARTESIAN_POINT('',(-39.9751670169646,-35.,5.));
#17539=CARTESIAN_POINT('Origin',(-39.9751670169646,-25.,5.));
#17540=CARTESIAN_POINT('',(-49.9751670169646,-25.,0.));
#17541=CARTESIAN_POINT('',(-49.9751670169646,-25.,1.25));
#17542=CARTESIAN_POINT('',(-39.9751670169646,-35.,0.));
#17543=CARTESIAN_POINT('Origin',(-39.9751670169646,-25.,0.));
#17544=CARTESIAN_POINT('',(-39.9751670169646,-35.,1.25));
#17545=CARTESIAN_POINT('Origin',(-49.9751670169646,0.,0.));
#17546=CARTESIAN_POINT('',(-49.9751670169646,0.,5.));
#17547=CARTESIAN_POINT('',(-49.9751670169646,0.,0.));
#17548=CARTESIAN_POINT('Origin',(-35.0075079285187,0.,5.));
#17549=CARTESIAN_POINT('',(-35.0075079285187,-19.5,5.));
#17550=CARTESIAN_POINT('',(-35.0075079285187,-25.,10.5));
#17551=CARTESIAN_POINT('Origin',(-35.0075079285187,-19.5,10.5));
#17552=CARTESIAN_POINT('',(-35.0075079285187,-25.,37.0308437753216));
#17553=CARTESIAN_POINT('',(-35.0075079285187,-25.,5.));
#17554=CARTESIAN_POINT('',(-35.0075079285187,-22.,37.0308437753216));
#17555=CARTESIAN_POINT('',(-35.0075079285187,0.,37.0308437753216));
#17556=CARTESIAN_POINT('',(-35.0075079285187,-22.,13.));
#17557=CARTESIAN_POINT('',(-35.0075079285187,-22.,18.7577109438304));
#17558=CARTESIAN_POINT('',(-35.0075079285187,-19.,10.));
#17559=CARTESIAN_POINT('Origin',(-35.0075079285187,-19.,13.));
#17560=CARTESIAN_POINT('',(-35.0075079285187,0.,10.));
#17561=CARTESIAN_POINT('',(-35.0075079285187,0.,5.));
#17562=CARTESIAN_POINT('Origin',(-19.9792411332937,0.,29.9773129029999));
#17563=CARTESIAN_POINT('',(-12.4213924902778,-25.,29.9773129029999));
#17564=CARTESIAN_POINT('Origin',(-19.9792411332937,-25.,29.9773129029999));
#17565=CARTESIAN_POINT('',(-12.4213924902778,-22.,29.9773129029999));
#17566=CARTESIAN_POINT('',(-12.4213924902778,0.,29.9773129029999));
#17567=CARTESIAN_POINT('Origin',(-19.9792411332937,-22.,29.9773129029999));
#17568=CARTESIAN_POINT('Origin',(-35.0075079285187,0.,37.0308437753216));
#17569=CARTESIAN_POINT('',(-27.0075079285187,-22.,45.0308437753216));
#17570=CARTESIAN_POINT('',(-33.010424909369,-22.,39.0279267944712));
#17571=CARTESIAN_POINT('',(-27.0075079285187,-25.,45.0308437753216));
#17572=CARTESIAN_POINT('',(-35.0075079285187,-25.,37.0308437753216));
#17573=CARTESIAN_POINT('',(-27.0075079285187,0.,45.0308437753216));
#17574=CARTESIAN_POINT('Origin',(39.9751670169646,-25.,1.25));
#17575=CARTESIAN_POINT('',(49.9751670169646,-25.,5.));
#17576=CARTESIAN_POINT('',(39.9751670169646,-35.,5.));
#17577=CARTESIAN_POINT('Origin',(39.9751670169646,-25.,5.));
#17578=CARTESIAN_POINT('',(39.9751670169646,-35.,0.));
#17579=CARTESIAN_POINT('',(39.9751670169646,-35.,1.25));
#17580=CARTESIAN_POINT('',(49.9751670169646,-25.,0.));
#17581=CARTESIAN_POINT('Origin',(39.9751670169646,-25.,0.));
#17582=CARTESIAN_POINT('',(49.9751670169646,-25.,1.25));
#17583=CARTESIAN_POINT('Origin',(24.9875835084823,-35.,2.5));
#17584=CARTESIAN_POINT('',(0.,-35.,5.));
#17585=CARTESIAN_POINT('',(0.,-35.,0.));
#17586=CARTESIAN_POINT('Origin',(49.9751670169646,0.,5.));
#17587=CARTESIAN_POINT('',(49.9751670169646,0.,5.));
#17588=CARTESIAN_POINT('',(35.0075079285187,-19.5,5.));
#17589=CARTESIAN_POINT('',(35.0075079285187,0.,5.));
#17590=CARTESIAN_POINT('',(8.75187698212967,-19.5,5.));
#17591=CARTESIAN_POINT('Origin',(49.9751670169646,0.,0.));
#17592=CARTESIAN_POINT('',(49.9751670169646,0.,0.));
#17593=CARTESIAN_POINT('Origin',(0.,0.,0.));
#17594=CARTESIAN_POINT('Origin',(26.255630946389,-19.,13.));
#17595=CARTESIAN_POINT('',(35.0075079285187,-22.,13.));
#17596=CARTESIAN_POINT('',(26.255630946389,-22.,13.));
#17597=CARTESIAN_POINT('',(35.0075079285187,-19.,10.));
#17598=CARTESIAN_POINT('Origin',(35.0075079285187,-19.,13.));
#17599=CARTESIAN_POINT('',(26.255630946389,-19.,10.));
#17600=CARTESIAN_POINT('Origin',(17.5037539642593,-22.,27.5154218876608));
#17601=CARTESIAN_POINT('',(27.0075079285187,-22.,45.0308437753216));
#17602=CARTESIAN_POINT('',(-22.255630946389,-22.,45.0308437753216));
#17603=CARTESIAN_POINT('',(35.0075079285187,-22.,37.0308437753216));
#17604=CARTESIAN_POINT('',(33.010424909369,-22.,39.0279267944712));
#17605=CARTESIAN_POINT('',(35.0075079285187,-22.,18.7577109438304));
#17606=CARTESIAN_POINT('',(12.4213924902778,-22.,29.9773129029999));
#17607=CARTESIAN_POINT('Origin',(19.9792411332937,-22.,29.9773129029999));
#17608=CARTESIAN_POINT('Origin',(8.75187698212967,-19.5,10.5));
#17609=CARTESIAN_POINT('',(35.0075079285187,-25.,10.5));
#17610=CARTESIAN_POINT('Origin',(35.0075079285187,-19.5,10.5));
#17611=CARTESIAN_POINT('',(8.75187698212967,-25.,10.5));
#17612=CARTESIAN_POINT('Origin',(17.5037539642593,-25.,7.5));
#17613=CARTESIAN_POINT('',(35.0075079285187,-25.,37.0308437753216));
#17614=CARTESIAN_POINT('',(35.0075079285187,-25.,5.));
#17615=CARTESIAN_POINT('',(27.0075079285187,-25.,45.0308437753216));
#17616=CARTESIAN_POINT('',(35.0075079285187,-25.,37.0308437753216));
#17617=CARTESIAN_POINT('',(27.0075079285187,-25.,45.0308437753216));
#17618=CARTESIAN_POINT('',(12.4213924902778,-25.,29.9773129029999));
#17619=CARTESIAN_POINT('Origin',(19.9792411332937,-25.,29.9773129029999));
#17620=CARTESIAN_POINT('Origin',(35.0075079285187,0.,5.));
#17621=CARTESIAN_POINT('',(35.0075079285187,0.,10.));
#17622=CARTESIAN_POINT('',(35.0075079285187,0.,37.0308437753216));
#17623=CARTESIAN_POINT('Origin',(19.9792411332937,0.,29.9773129029999));
#17624=CARTESIAN_POINT('',(12.4213924902778,0.,29.9773129029999));
#17625=CARTESIAN_POINT('Origin',(27.0075079285187,0.,45.0308437753216));
#17626=CARTESIAN_POINT('',(27.0075079285187,0.,45.0308437753216));
#17627=CARTESIAN_POINT('Origin',(35.0075079285187,0.,37.0308437753216));
#17628=CARTESIAN_POINT('Origin',(35.0075079285187,0.,10.));
#279246=UNCERTAINTY_MEASURE_WITH_UNIT(LENGTH_MEASURE(0.01),#279267,
'DISTANCE_ACCURACY_VALUE',
'Maximum model space distance between geometric entities at asserted c
onnectivities');
#279255=UNCERTAINTY_MEASURE_WITH_UNIT(LENGTH_MEASURE(0.01),#279267,
'DISTANCE_ACCURACY_VALUE',
'Maximum model space distance between geometric entities at asserted c
onnectivities');
#279257=(
GEOMETRIC_REPRESENTATION_CONTEXT(3)
GLOBAL_UNCERTAINTY_ASSIGNED_CONTEXT((#279246))
GLOBAL_UNIT_ASSIGNED_CONTEXT((#279267,#279269,#279270))
REPRESENTATION_CONTEXT('','3D')
);
#279266=(
GEOMETRIC_REPRESENTATION_CONTEXT(3)
GLOBAL_UNCERTAINTY_ASSIGNED_CONTEXT((#279255))
GLOBAL_UNIT_ASSIGNED_CONTEXT((#279267,#279269,#279270))
REPRESENTATION_CONTEXT('','3D')
);
#279267=(
LENGTH_UNIT()
NAMED_UNIT(*)
SI_UNIT(.MILLI.,.METRE.)
);
#279269=(
NAMED_UNIT(*)
PLANE_ANGLE_UNIT()
SI_UNIT($,.RADIAN.)
);
#279270=(
NAMED_UNIT(*)
SI_UNIT($,.STERADIAN.)
SOLID_ANGLE_UNIT()
);
#279272=SHAPE_DEFINITION_REPRESENTATION(#279282,#279301);
#279282=PRODUCT_DEFINITION_SHAPE('',$,#279312);
#279301=SHAPE_REPRESENTATION('',(#15048),#279257);
#279310=PRODUCT_DEFINITION_CONTEXT('part definition',#279342,'design');
#279312=PRODUCT_DEFINITION('base','Base',#279322,#279310);
#279322=PRODUCT_DEFINITION_FORMATION('',$,#279345);
#279342=APPLICATION_CONTEXT(
'Core Data for Automotive Mechanical Design Process');
#279343=PRODUCT_CONTEXT('part definition',#279342,'mechanical');
#279345=PRODUCT('base','Base',$,(#279343));
#279355=PRESENTATION_STYLE_ASSIGNMENT((#279357));
#279357=SURFACE_STYLE_USAGE(.BOTH.,#279359);
#279359=SURFACE_SIDE_STYLE('',(#279361));
#279361=SURFACE_STYLE_FILL_AREA(#279363);
#279363=FILL_AREA_STYLE('Opaque(160,160,160)',(#279365));
#279365=FILL_AREA_STYLE_COLOUR('Opaque(160,160,160)',#279367);
#279367=COLOUR_RGB('Opaque(160,160,160)', 0.66274510, 0.83137255, 0.94901961);
ENDSEC;
END-ISO-10303-21;
